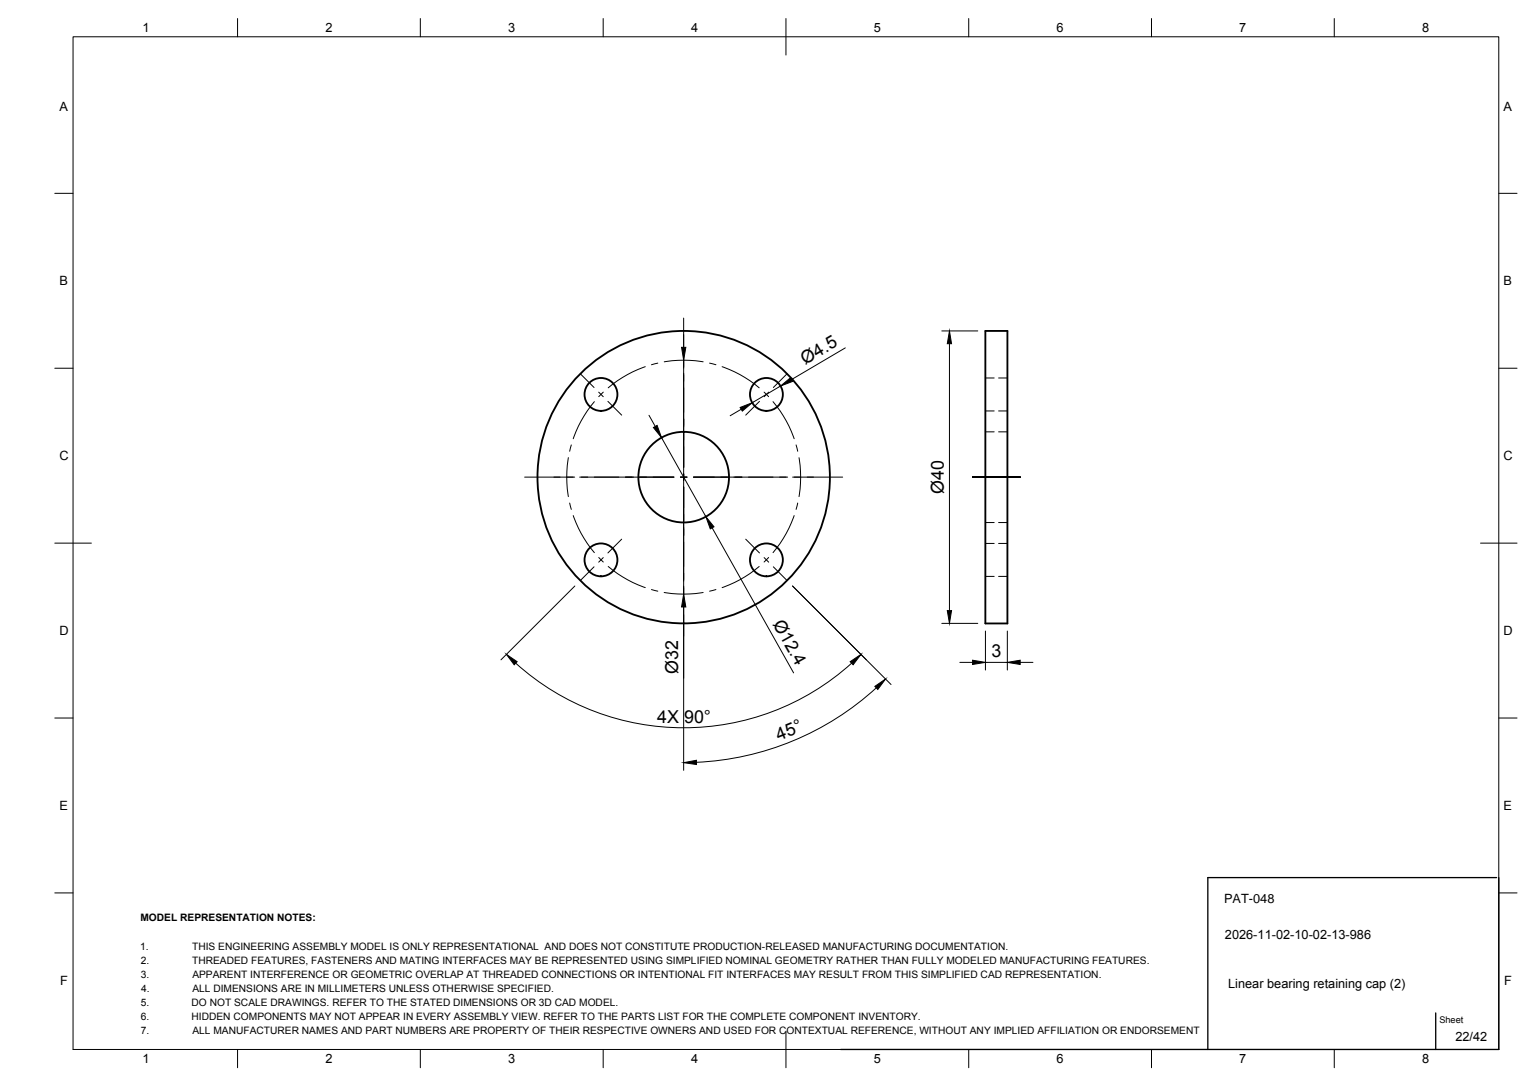
ISO-10303-21;
HEADER;
/* Generated by software containing ST-Developer
 * from STEP Tools, Inc. (www.steptools.com) 
 */

FILE_DESCRIPTION(
/* description */ ('Guided pneumatic stop gate'),
/* implementation_level */ '2;1');

FILE_NAME(
/* name */ 'Linear bearing retaining cap (2).step',
/* time_stamp */ '2026-10-27T21:43:45-07:00',
/* author */ (''),
/* organization */ (''),
/* preprocessor_version */ 'ST-DEVELOPER v20.2',
/* originating_system */ 'Autodesk Translation Framework v15.17.0.0',
/* authorisation */ '');

FILE_SCHEMA (('AUTOMOTIVE_DESIGN { 1 0 10303 214 3 1 1 }'));
ENDSEC;

DATA;
#10=MECHANICAL_DESIGN_GEOMETRIC_PRESENTATION_REPRESENTATION('',(#557),#14392);
#473=SHAPE_REPRESENTATION_RELATIONSHIP('SRR','None',#14608,#515);
#515=ADVANCED_BREP_SHAPE_REPRESENTATION('',(#598),#14370);
#557=STYLED_ITEM('',(#14891),#598);
#598=MANIFOLD_SOLID_BREP('Body1',#7898);
#757=FACE_BOUND('',#2024,.T.);
#758=FACE_BOUND('',#2025,.T.);
#759=FACE_BOUND('',#2026,.T.);
#760=FACE_BOUND('',#2027,.T.);
#761=FACE_BOUND('',#2028,.T.);
#762=FACE_BOUND('',#2030,.T.);
#763=FACE_BOUND('',#2031,.T.);
#764=FACE_BOUND('',#2032,.T.);
#765=FACE_BOUND('',#2033,.T.);
#766=FACE_BOUND('',#2034,.T.);
#999=PLANE('',#8957);
#1000=PLANE('',#8958);
#1400=FACE_OUTER_BOUND('',#2017,.T.);
#1401=FACE_OUTER_BOUND('',#2018,.T.);
#1402=FACE_OUTER_BOUND('',#2019,.T.);
#1403=FACE_OUTER_BOUND('',#2020,.T.);
#1404=FACE_OUTER_BOUND('',#2021,.T.);
#1405=FACE_OUTER_BOUND('',#2022,.T.);
#1406=FACE_OUTER_BOUND('',#2023,.T.);
#1407=FACE_OUTER_BOUND('',#2029,.T.);
#2017=EDGE_LOOP('',(#6474,#6475,#6476,#6477));
#2018=EDGE_LOOP('',(#6478,#6479,#6480,#6481));
#2019=EDGE_LOOP('',(#6482,#6483,#6484,#6485));
#2020=EDGE_LOOP('',(#6486,#6487,#6488,#6489));
#2021=EDGE_LOOP('',(#6490,#6491,#6492,#6493));
#2022=EDGE_LOOP('',(#6494,#6495,#6496,#6497));
#2023=EDGE_LOOP('',(#6498));
#2024=EDGE_LOOP('',(#6499));
#2025=EDGE_LOOP('',(#6500));
#2026=EDGE_LOOP('',(#6501));
#2027=EDGE_LOOP('',(#6502));
#2028=EDGE_LOOP('',(#6503));
#2029=EDGE_LOOP('',(#6504));
#2030=EDGE_LOOP('',(#6505));
#2031=EDGE_LOOP('',(#6506));
#2032=EDGE_LOOP('',(#6507));
#2033=EDGE_LOOP('',(#6508));
#2034=EDGE_LOOP('',(#6509));
#2600=LINE('',#13208,#3145);
#2601=LINE('',#13214,#3146);
#2602=LINE('',#13220,#3147);
#2603=LINE('',#13226,#3148);
#2604=LINE('',#13232,#3149);
#2605=LINE('',#13238,#3150);
#3145=VECTOR('',#10817,0.225);
#3146=VECTOR('',#10824,0.225);
#3147=VECTOR('',#10831,0.225);
#3148=VECTOR('',#10838,0.225);
#3149=VECTOR('',#10845,0.62);
#3150=VECTOR('',#10852,2.);
#3599=CIRCLE('',#8940,0.225);
#3600=CIRCLE('',#8941,0.225);
#3601=CIRCLE('',#8943,0.225);
#3602=CIRCLE('',#8944,0.225);
#3603=CIRCLE('',#8946,0.225);
#3604=CIRCLE('',#8947,0.225);
#3605=CIRCLE('',#8949,0.225);
#3606=CIRCLE('',#8950,0.225);
#3607=CIRCLE('',#8952,0.62);
#3608=CIRCLE('',#8953,0.62);
#3609=CIRCLE('',#8955,2.);
#3610=CIRCLE('',#8956,2.);
#4108=VERTEX_POINT('',#13205);
#4109=VERTEX_POINT('',#13207);
#4110=VERTEX_POINT('',#13211);
#4111=VERTEX_POINT('',#13213);
#4112=VERTEX_POINT('',#13217);
#4113=VERTEX_POINT('',#13219);
#4114=VERTEX_POINT('',#13223);
#4115=VERTEX_POINT('',#13225);
#4116=VERTEX_POINT('',#13229);
#4117=VERTEX_POINT('',#13231);
#4118=VERTEX_POINT('',#13235);
#4119=VERTEX_POINT('',#13237);
#4935=EDGE_CURVE('',#4108,#4108,#3599,.T.);
#4936=EDGE_CURVE('',#4108,#4109,#2600,.T.);
#4937=EDGE_CURVE('',#4109,#4109,#3600,.T.);
#4938=EDGE_CURVE('',#4110,#4110,#3601,.T.);
#4939=EDGE_CURVE('',#4110,#4111,#2601,.T.);
#4940=EDGE_CURVE('',#4111,#4111,#3602,.T.);
#4941=EDGE_CURVE('',#4112,#4112,#3603,.T.);
#4942=EDGE_CURVE('',#4112,#4113,#2602,.T.);
#4943=EDGE_CURVE('',#4113,#4113,#3604,.T.);
#4944=EDGE_CURVE('',#4114,#4114,#3605,.T.);
#4945=EDGE_CURVE('',#4114,#4115,#2603,.T.);
#4946=EDGE_CURVE('',#4115,#4115,#3606,.T.);
#4947=EDGE_CURVE('',#4116,#4116,#3607,.T.);
#4948=EDGE_CURVE('',#4116,#4117,#2604,.T.);
#4949=EDGE_CURVE('',#4117,#4117,#3608,.T.);
#4950=EDGE_CURVE('',#4118,#4118,#3609,.T.);
#4951=EDGE_CURVE('',#4118,#4119,#2605,.T.);
#4952=EDGE_CURVE('',#4119,#4119,#3610,.T.);
#6474=ORIENTED_EDGE('',*,*,#4935,.F.);
#6475=ORIENTED_EDGE('',*,*,#4936,.T.);
#6476=ORIENTED_EDGE('',*,*,#4937,.F.);
#6477=ORIENTED_EDGE('',*,*,#4936,.F.);
#6478=ORIENTED_EDGE('',*,*,#4938,.F.);
#6479=ORIENTED_EDGE('',*,*,#4939,.T.);
#6480=ORIENTED_EDGE('',*,*,#4940,.F.);
#6481=ORIENTED_EDGE('',*,*,#4939,.F.);
#6482=ORIENTED_EDGE('',*,*,#4941,.F.);
#6483=ORIENTED_EDGE('',*,*,#4942,.T.);
#6484=ORIENTED_EDGE('',*,*,#4943,.F.);
#6485=ORIENTED_EDGE('',*,*,#4942,.F.);
#6486=ORIENTED_EDGE('',*,*,#4944,.F.);
#6487=ORIENTED_EDGE('',*,*,#4945,.T.);
#6488=ORIENTED_EDGE('',*,*,#4946,.F.);
#6489=ORIENTED_EDGE('',*,*,#4945,.F.);
#6490=ORIENTED_EDGE('',*,*,#4947,.F.);
#6491=ORIENTED_EDGE('',*,*,#4948,.T.);
#6492=ORIENTED_EDGE('',*,*,#4949,.T.);
#6493=ORIENTED_EDGE('',*,*,#4948,.F.);
#6494=ORIENTED_EDGE('',*,*,#4950,.F.);
#6495=ORIENTED_EDGE('',*,*,#4951,.T.);
#6496=ORIENTED_EDGE('',*,*,#4952,.T.);
#6497=ORIENTED_EDGE('',*,*,#4951,.F.);
#6498=ORIENTED_EDGE('',*,*,#4950,.T.);
#6499=ORIENTED_EDGE('',*,*,#4947,.T.);
#6500=ORIENTED_EDGE('',*,*,#4946,.T.);
#6501=ORIENTED_EDGE('',*,*,#4943,.T.);
#6502=ORIENTED_EDGE('',*,*,#4940,.T.);
#6503=ORIENTED_EDGE('',*,*,#4937,.T.);
#6504=ORIENTED_EDGE('',*,*,#4952,.F.);
#6505=ORIENTED_EDGE('',*,*,#4949,.F.);
#6506=ORIENTED_EDGE('',*,*,#4944,.T.);
#6507=ORIENTED_EDGE('',*,*,#4941,.T.);
#6508=ORIENTED_EDGE('',*,*,#4938,.T.);
#6509=ORIENTED_EDGE('',*,*,#4935,.T.);
#7345=CYLINDRICAL_SURFACE('',#8939,0.225);
#7346=CYLINDRICAL_SURFACE('',#8942,0.225);
#7347=CYLINDRICAL_SURFACE('',#8945,0.225);
#7348=CYLINDRICAL_SURFACE('',#8948,0.225);
#7349=CYLINDRICAL_SURFACE('',#8951,0.62);
#7350=CYLINDRICAL_SURFACE('',#8954,2.);
#7682=ADVANCED_FACE('',(#1400),#7345,.F.);
#7683=ADVANCED_FACE('',(#1401),#7346,.F.);
#7684=ADVANCED_FACE('',(#1402),#7347,.F.);
#7685=ADVANCED_FACE('',(#1403),#7348,.F.);
#7686=ADVANCED_FACE('',(#1404),#7349,.F.);
#7687=ADVANCED_FACE('',(#1405),#7350,.T.);
#7688=ADVANCED_FACE('',(#1406,#757,#758,#759,#760,#761),#999,.T.);
#7689=ADVANCED_FACE('',(#1407,#762,#763,#764,#765,#766),#1000,.F.);
#7898=CLOSED_SHELL('',(#7682,#7683,#7684,#7685,#7686,#7687,#7688,#7689));
#8938=AXIS2_PLACEMENT_3D('',#13203,#10811,#10812);
#8939=AXIS2_PLACEMENT_3D('',#13204,#10813,#10814);
#8940=AXIS2_PLACEMENT_3D('',#13206,#10815,#10816);
#8941=AXIS2_PLACEMENT_3D('',#13209,#10818,#10819);
#8942=AXIS2_PLACEMENT_3D('',#13210,#10820,#10821);
#8943=AXIS2_PLACEMENT_3D('',#13212,#10822,#10823);
#8944=AXIS2_PLACEMENT_3D('',#13215,#10825,#10826);
#8945=AXIS2_PLACEMENT_3D('',#13216,#10827,#10828);
#8946=AXIS2_PLACEMENT_3D('',#13218,#10829,#10830);
#8947=AXIS2_PLACEMENT_3D('',#13221,#10832,#10833);
#8948=AXIS2_PLACEMENT_3D('',#13222,#10834,#10835);
#8949=AXIS2_PLACEMENT_3D('',#13224,#10836,#10837);
#8950=AXIS2_PLACEMENT_3D('',#13227,#10839,#10840);
#8951=AXIS2_PLACEMENT_3D('',#13228,#10841,#10842);
#8952=AXIS2_PLACEMENT_3D('',#13230,#10843,#10844);
#8953=AXIS2_PLACEMENT_3D('',#13233,#10846,#10847);
#8954=AXIS2_PLACEMENT_3D('',#13234,#10848,#10849);
#8955=AXIS2_PLACEMENT_3D('',#13236,#10850,#10851);
#8956=AXIS2_PLACEMENT_3D('',#13239,#10853,#10854);
#8957=AXIS2_PLACEMENT_3D('',#13240,#10855,#10856);
#8958=AXIS2_PLACEMENT_3D('',#13241,#10857,#10858);
#10811=DIRECTION('axis',(0.,0.,1.));
#10812=DIRECTION('refdir',(1.,0.,0.));
#10813=DIRECTION('center_axis',(0.,1.,0.));
#10814=DIRECTION('ref_axis',(1.,0.,0.));
#10815=DIRECTION('center_axis',(0.,1.,0.));
#10816=DIRECTION('ref_axis',(1.,0.,0.));
#10817=DIRECTION('',(0.,1.,0.));
#10818=DIRECTION('center_axis',(0.,-1.,0.));
#10819=DIRECTION('ref_axis',(1.,0.,0.));
#10820=DIRECTION('center_axis',(0.,1.,0.));
#10821=DIRECTION('ref_axis',(1.,0.,0.));
#10822=DIRECTION('center_axis',(0.,1.,0.));
#10823=DIRECTION('ref_axis',(1.,0.,0.));
#10824=DIRECTION('',(0.,1.,0.));
#10825=DIRECTION('center_axis',(0.,-1.,0.));
#10826=DIRECTION('ref_axis',(1.,0.,0.));
#10827=DIRECTION('center_axis',(0.,1.,0.));
#10828=DIRECTION('ref_axis',(1.,0.,0.));
#10829=DIRECTION('center_axis',(0.,1.,0.));
#10830=DIRECTION('ref_axis',(1.,0.,0.));
#10831=DIRECTION('',(0.,1.,0.));
#10832=DIRECTION('center_axis',(0.,-1.,0.));
#10833=DIRECTION('ref_axis',(1.,0.,0.));
#10834=DIRECTION('center_axis',(0.,1.,0.));
#10835=DIRECTION('ref_axis',(1.,0.,0.));
#10836=DIRECTION('center_axis',(0.,1.,0.));
#10837=DIRECTION('ref_axis',(1.,0.,0.));
#10838=DIRECTION('',(0.,1.,0.));
#10839=DIRECTION('center_axis',(0.,-1.,0.));
#10840=DIRECTION('ref_axis',(1.,0.,0.));
#10841=DIRECTION('center_axis',(0.,1.,0.));
#10842=DIRECTION('ref_axis',(1.,0.,0.));
#10843=DIRECTION('center_axis',(0.,-1.,0.));
#10844=DIRECTION('ref_axis',(1.,0.,0.));
#10845=DIRECTION('',(0.,-1.,0.));
#10846=DIRECTION('center_axis',(0.,-1.,0.));
#10847=DIRECTION('ref_axis',(1.,0.,0.));
#10848=DIRECTION('center_axis',(0.,1.,0.));
#10849=DIRECTION('ref_axis',(1.,0.,0.));
#10850=DIRECTION('center_axis',(0.,1.,0.));
#10851=DIRECTION('ref_axis',(1.,0.,0.));
#10852=DIRECTION('',(0.,-1.,0.));
#10853=DIRECTION('center_axis',(0.,1.,0.));
#10854=DIRECTION('ref_axis',(1.,0.,0.));
#10855=DIRECTION('center_axis',(0.,1.,0.));
#10856=DIRECTION('ref_axis',(1.,0.,0.));
#10857=DIRECTION('center_axis',(0.,1.,0.));
#10858=DIRECTION('ref_axis',(1.,0.,0.));
#13203=CARTESIAN_POINT('',(0.,0.,0.));
#13204=CARTESIAN_POINT('Origin',(3.86862915010152,5.6,3.36862915010152));
#13205=CARTESIAN_POINT('',(3.64362915010152,5.7,3.36862915010152));
#13206=CARTESIAN_POINT('Origin',(3.86862915010152,5.7,3.36862915010152));
#13207=CARTESIAN_POINT('',(3.64362915010152,6.,3.36862915010152));
#13208=CARTESIAN_POINT('',(3.64362915010152,5.6,3.36862915010152));
#13209=CARTESIAN_POINT('Origin',(3.86862915010152,6.,3.36862915010152));
#13210=CARTESIAN_POINT('Origin',(3.86862915010152,5.6,5.63137084989848));
#13211=CARTESIAN_POINT('',(3.64362915010152,5.7,5.63137084989848));
#13212=CARTESIAN_POINT('Origin',(3.86862915010152,5.7,5.63137084989848));
#13213=CARTESIAN_POINT('',(3.64362915010152,6.,5.63137084989848));
#13214=CARTESIAN_POINT('',(3.64362915010152,5.6,5.63137084989848));
#13215=CARTESIAN_POINT('Origin',(3.86862915010152,6.,5.63137084989848));
#13216=CARTESIAN_POINT('Origin',(6.13137084989848,5.6,5.63137084989848));
#13217=CARTESIAN_POINT('',(5.90637084989848,5.7,5.63137084989848));
#13218=CARTESIAN_POINT('Origin',(6.13137084989848,5.7,5.63137084989848));
#13219=CARTESIAN_POINT('',(5.90637084989848,6.,5.63137084989848));
#13220=CARTESIAN_POINT('',(5.90637084989848,5.6,5.63137084989848));
#13221=CARTESIAN_POINT('Origin',(6.13137084989848,6.,5.63137084989848));
#13222=CARTESIAN_POINT('Origin',(6.13137084989848,5.6,3.36862915010152));
#13223=CARTESIAN_POINT('',(5.90637084989848,5.7,3.36862915010152));
#13224=CARTESIAN_POINT('Origin',(6.13137084989848,5.7,3.36862915010152));
#13225=CARTESIAN_POINT('',(5.90637084989848,6.,3.36862915010152));
#13226=CARTESIAN_POINT('',(5.90637084989848,5.6,3.36862915010152));
#13227=CARTESIAN_POINT('Origin',(6.13137084989848,6.,3.36862915010152));
#13228=CARTESIAN_POINT('Origin',(5.,5.7,4.5));
#13229=CARTESIAN_POINT('',(4.38,6.,4.5));
#13230=CARTESIAN_POINT('Origin',(5.,6.,4.5));
#13231=CARTESIAN_POINT('',(4.38,5.7,4.5));
#13232=CARTESIAN_POINT('',(4.38,5.7,4.5));
#13233=CARTESIAN_POINT('Origin',(5.,5.7,4.5));
#13234=CARTESIAN_POINT('Origin',(5.,5.7,4.5));
#13235=CARTESIAN_POINT('',(3.,6.,4.5));
#13236=CARTESIAN_POINT('Origin',(5.,6.,4.5));
#13237=CARTESIAN_POINT('',(3.,5.7,4.5));
#13238=CARTESIAN_POINT('',(3.,5.7,4.5));
#13239=CARTESIAN_POINT('Origin',(5.,5.7,4.5));
#13240=CARTESIAN_POINT('Origin',(5.,6.,4.5));
#13241=CARTESIAN_POINT('Origin',(5.,5.7,4.5));
#14322=UNCERTAINTY_MEASURE_WITH_UNIT(LENGTH_MEASURE(0.001),#14393,
'DISTANCE_ACCURACY_VALUE',
'Maximum model space distance between geometric entities at asserted c
onnectivities');
#14344=UNCERTAINTY_MEASURE_WITH_UNIT(LENGTH_MEASURE(0.001),#14393,
'DISTANCE_ACCURACY_VALUE',
'Maximum model space distance between geometric entities at asserted c
onnectivities');
#14370=(
GEOMETRIC_REPRESENTATION_CONTEXT(3)
GLOBAL_UNCERTAINTY_ASSIGNED_CONTEXT((#14322))
GLOBAL_UNIT_ASSIGNED_CONTEXT((#14393,#14395,#14396))
REPRESENTATION_CONTEXT('','3D')
);
#14392=(
GEOMETRIC_REPRESENTATION_CONTEXT(3)
GLOBAL_UNCERTAINTY_ASSIGNED_CONTEXT((#14344))
GLOBAL_UNIT_ASSIGNED_CONTEXT((#14393,#14395,#14396))
REPRESENTATION_CONTEXT('','3D')
);
#14393=(
LENGTH_UNIT()
NAMED_UNIT(*)
SI_UNIT(.CENTI.,.METRE.)
);
#14395=(
NAMED_UNIT(*)
PLANE_ANGLE_UNIT()
SI_UNIT($,.RADIAN.)
);
#14396=(
NAMED_UNIT(*)
SI_UNIT($,.STERADIAN.)
SOLID_ANGLE_UNIT()
);
#14422=SHAPE_DEFINITION_REPRESENTATION(#14471,#14608);
#14471=PRODUCT_DEFINITION_SHAPE('',$,#14656);
#14608=SHAPE_REPRESENTATION('',(#8938),#14370);
#14630=PRODUCT_DEFINITION_CONTEXT('part definition',#14773,'design');
#14656=PRODUCT_DEFINITION('Linear bearing retaining cap (2)',
'Linear bearing retaining cap (2)',#14703,#14630);
#14703=PRODUCT_DEFINITION_FORMATION('',$,#14800);
#14773=APPLICATION_CONTEXT(
'Core Data for Automotive Mechanical Design Process');
#14774=PRODUCT_CONTEXT('part definition',#14773,'mechanical');
#14800=PRODUCT('Linear bearing retaining cap (2)',
'Linear bearing retaining cap (2)','Linear bearing retaining cap (2)',(#14774));
#14885=COLOUR_RGB('Grey',0.48,0.52,0.57);
#14886=FILL_AREA_STYLE_COLOUR('',#14885);
#14887=FILL_AREA_STYLE('',(#14886));
#14888=SURFACE_STYLE_FILL_AREA(#14887);
#14889=SURFACE_SIDE_STYLE('',(#14888));
#14890=SURFACE_STYLE_USAGE(.BOTH.,#14889);
#14891=PRESENTATION_STYLE_ASSIGNMENT((#14890));
ENDSEC;
END-ISO-10303-21;
